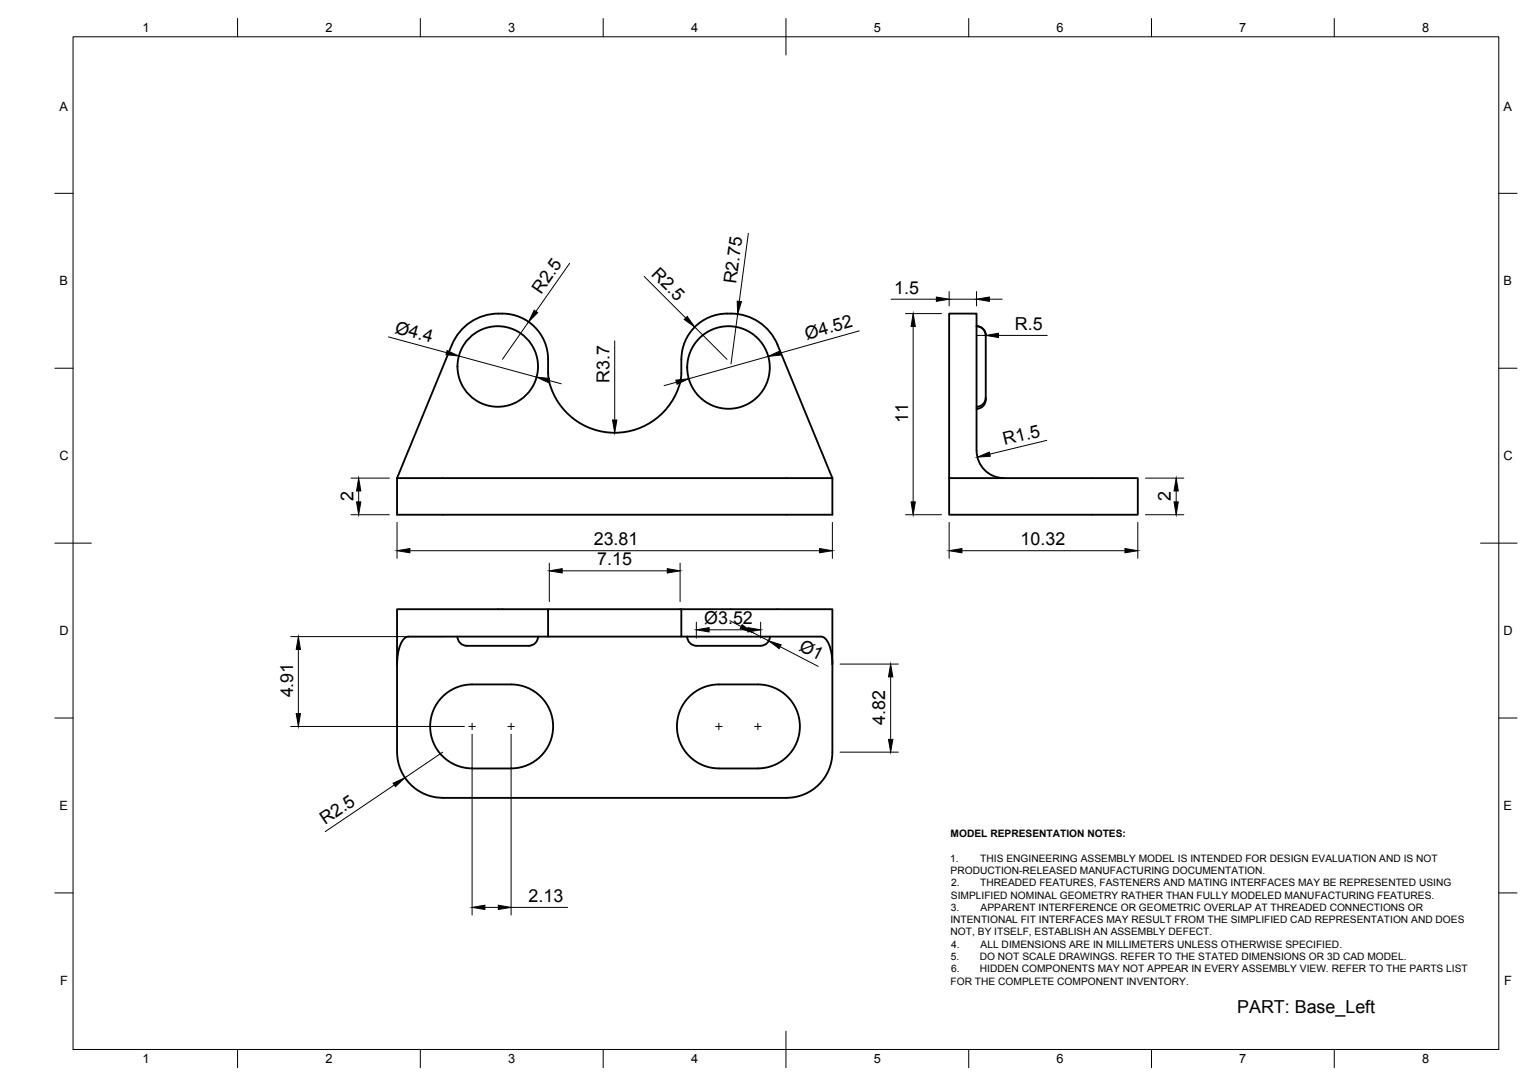
ISO-10303-21;
HEADER;
/* Generated by software containing ST-Developer
 * from STEP Tools, Inc. (www.steptools.com) 
 */

FILE_DESCRIPTION(
/* description */ (''),
/* implementation_level */ '2;1');

FILE_NAME(
/* name */ 'Base_Left.step',
/* time_stamp */ '2026-10-05T16:20:14-07:00',
/* author */ (''),
/* organization */ (''),
/* preprocessor_version */ 'ST-DEVELOPER v20.2',
/* originating_system */ 'Autodesk Translation Framework v15.15.0.0',
/* authorisation */ '');

FILE_SCHEMA (('AUTOMOTIVE_DESIGN { 1 0 10303 214 3 1 1 }'));
ENDSEC;

DATA;
#10=MECHANICAL_DESIGN_GEOMETRIC_PRESENTATION_REPRESENTATION('',(#248),#23577);
#207=ELLIPSE('',#4296,1.6218841056004,1.5);
#208=ELLIPSE('',#4297,1.6218841056004,1.5);
#213=TOROIDAL_SURFACE('',#4285,1.70133516896762,0.5);
#214=TOROIDAL_SURFACE('',#4290,1.75974879114541,0.5);
#230=SHAPE_REPRESENTATION_RELATIONSHIP('SRR','None',#23613,#239);
#239=ADVANCED_BREP_SHAPE_REPRESENTATION('',(#257),#23569);
#248=STYLED_ITEM('',(#23666),#257);
#257=MANIFOLD_SOLID_BREP('Body1',#4158);
#269=FACE_BOUND('',#640,.T.);
#270=FACE_BOUND('',#641,.T.);
#271=FACE_BOUND('',#670,.T.);
#272=FACE_BOUND('',#671,.T.);
#273=FACE_BOUND('',#673,.T.);
#274=FACE_BOUND('',#674,.T.);
#304=PLANE('',#4289);
#305=PLANE('',#4294);
#306=PLANE('',#4298);
#307=PLANE('',#4308);
#308=PLANE('',#4311);
#309=PLANE('',#4314);
#310=PLANE('',#4317);
#311=PLANE('',#4320);
#312=PLANE('',#4325);
#313=PLANE('',#4326);
#314=PLANE('',#4327);
#315=PLANE('',#4328);
#316=PLANE('',#4332);
#317=PLANE('',#4336);
#318=PLANE('',#4340);
#319=PLANE('',#4344);
#320=PLANE('',#4348);
#321=PLANE('',#4352);
#322=PLANE('',#4353);
#404=FACE_OUTER_BOUND('',#634,.T.);
#405=FACE_OUTER_BOUND('',#635,.T.);
#406=FACE_OUTER_BOUND('',#636,.T.);
#407=FACE_OUTER_BOUND('',#637,.T.);
#408=FACE_OUTER_BOUND('',#638,.T.);
#409=FACE_OUTER_BOUND('',#639,.T.);
#410=FACE_OUTER_BOUND('',#642,.T.);
#411=FACE_OUTER_BOUND('',#643,.T.);
#412=FACE_OUTER_BOUND('',#644,.T.);
#413=FACE_OUTER_BOUND('',#645,.T.);
#414=FACE_OUTER_BOUND('',#646,.T.);
#415=FACE_OUTER_BOUND('',#647,.T.);
#416=FACE_OUTER_BOUND('',#648,.T.);
#417=FACE_OUTER_BOUND('',#649,.T.);
#418=FACE_OUTER_BOUND('',#650,.T.);
#419=FACE_OUTER_BOUND('',#651,.T.);
#420=FACE_OUTER_BOUND('',#652,.T.);
#421=FACE_OUTER_BOUND('',#653,.T.);
#422=FACE_OUTER_BOUND('',#654,.T.);
#423=FACE_OUTER_BOUND('',#655,.T.);
#424=FACE_OUTER_BOUND('',#656,.T.);
#425=FACE_OUTER_BOUND('',#657,.T.);
#426=FACE_OUTER_BOUND('',#658,.T.);
#427=FACE_OUTER_BOUND('',#659,.T.);
#428=FACE_OUTER_BOUND('',#660,.T.);
#429=FACE_OUTER_BOUND('',#661,.T.);
#430=FACE_OUTER_BOUND('',#662,.T.);
#431=FACE_OUTER_BOUND('',#663,.T.);
#432=FACE_OUTER_BOUND('',#664,.T.);
#433=FACE_OUTER_BOUND('',#665,.T.);
#434=FACE_OUTER_BOUND('',#666,.T.);
#435=FACE_OUTER_BOUND('',#667,.T.);
#436=FACE_OUTER_BOUND('',#668,.T.);
#437=FACE_OUTER_BOUND('',#669,.T.);
#438=FACE_OUTER_BOUND('',#672,.T.);
#634=EDGE_LOOP('',(#2673,#2674,#2675,#2676));
#635=EDGE_LOOP('',(#2677));
#636=EDGE_LOOP('',(#2678,#2679,#2680,#2681));
#637=EDGE_LOOP('',(#2682));
#638=EDGE_LOOP('',(#2683,#2684,#2685,#2686));
#639=EDGE_LOOP('',(#2687,#2688,#2689,#2690,#2691,#2692,#2693,#2694,#2695,
#2696,#2697,#2698,#2699,#2700));
#640=EDGE_LOOP('',(#2701));
#641=EDGE_LOOP('',(#2702));
#642=EDGE_LOOP('',(#2703,#2704,#2705,#2706));
#643=EDGE_LOOP('',(#2707,#2708,#2709,#2710));
#644=EDGE_LOOP('',(#2711,#2712,#2713,#2714));
#645=EDGE_LOOP('',(#2715,#2716,#2717,#2718));
#646=EDGE_LOOP('',(#2719,#2720,#2721,#2722));
#647=EDGE_LOOP('',(#2723,#2724,#2725,#2726,#2727));
#648=EDGE_LOOP('',(#2728,#2729,#2730,#2731));
#649=EDGE_LOOP('',(#2732,#2733,#2734,#2735,#2736));
#650=EDGE_LOOP('',(#2737,#2738,#2739,#2740));
#651=EDGE_LOOP('',(#2741,#2742,#2743,#2744));
#652=EDGE_LOOP('',(#2745,#2746,#2747,#2748));
#653=EDGE_LOOP('',(#2749,#2750,#2751,#2752));
#654=EDGE_LOOP('',(#2753,#2754,#2755,#2756,#2757));
#655=EDGE_LOOP('',(#2758,#2759,#2760,#2761,#2762,#2763,#2764,#2765,#2766,
#2767,#2768,#2769,#2770,#2771,#2772,#2773));
#656=EDGE_LOOP('',(#2774,#2775,#2776,#2777));
#657=EDGE_LOOP('',(#2778,#2779,#2780,#2781));
#658=EDGE_LOOP('',(#2782,#2783,#2784,#2785));
#659=EDGE_LOOP('',(#2786,#2787,#2788,#2789));
#660=EDGE_LOOP('',(#2790,#2791,#2792,#2793));
#661=EDGE_LOOP('',(#2794,#2795,#2796,#2797));
#662=EDGE_LOOP('',(#2798,#2799,#2800,#2801));
#663=EDGE_LOOP('',(#2802,#2803,#2804,#2805));
#664=EDGE_LOOP('',(#2806,#2807,#2808,#2809));
#665=EDGE_LOOP('',(#2810,#2811,#2812,#2813,#2814));
#666=EDGE_LOOP('',(#2815,#2816,#2817,#2818));
#667=EDGE_LOOP('',(#2819,#2820,#2821,#2822));
#668=EDGE_LOOP('',(#2823,#2824,#2825,#2826));
#669=EDGE_LOOP('',(#2827,#2828,#2829,#2830,#2831,#2832));
#670=EDGE_LOOP('',(#2833,#2834,#2835,#2836));
#671=EDGE_LOOP('',(#2837,#2838,#2839,#2840));
#672=EDGE_LOOP('',(#2841,#2842,#2843,#2844,#2845,#2846));
#673=EDGE_LOOP('',(#2847,#2848,#2849,#2850));
#674=EDGE_LOOP('',(#2851,#2852,#2853,#2854));
#893=LINE('',#5835,#1178);
#894=LINE('',#5838,#1179);
#895=LINE('',#5841,#1180);
#896=LINE('',#5845,#1181);
#897=LINE('',#5849,#1182);
#898=LINE('',#5857,#1183);
#899=LINE('',#5861,#1184);
#900=LINE('',#5864,#1185);
#901=LINE('',#5867,#1186);
#902=LINE('',#5870,#1187);
#903=LINE('',#5873,#1188);
#904=LINE('',#5874,#1189);
#905=LINE('',#5879,#1190);
#906=LINE('',#5880,#1191);
#907=LINE('',#5883,#1192);
#908=LINE('',#5884,#1193);
#909=LINE('',#5888,#1194);
#910=LINE('',#5891,#1195);
#911=LINE('',#5892,#1196);
#912=LINE('',#5895,#1197);
#913=LINE('',#5898,#1198);
#914=LINE('',#5901,#1199);
#915=LINE('',#5902,#1200);
#916=LINE('',#5907,#1201);
#917=LINE('',#5908,#1202);
#918=LINE('',#5910,#1203);
#919=LINE('',#5914,#1204);
#920=LINE('',#5919,#1205);
#921=LINE('',#5921,#1206);
#922=LINE('',#5923,#1207);
#923=LINE('',#5924,#1208);
#924=LINE('',#5927,#1209);
#925=LINE('',#5928,#1210);
#926=LINE('',#5929,#1211);
#927=LINE('',#5934,#1212);
#928=LINE('',#5936,#1213);
#929=LINE('',#5938,#1214);
#930=LINE('',#5939,#1215);
#931=LINE('',#5945,#1216);
#932=LINE('',#5948,#1217);
#933=LINE('',#5950,#1218);
#934=LINE('',#5951,#1219);
#935=LINE('',#5958,#1220);
#936=LINE('',#5960,#1221);
#937=LINE('',#5962,#1222);
#938=LINE('',#5963,#1223);
#939=LINE('',#5969,#1224);
#940=LINE('',#5972,#1225);
#941=LINE('',#5974,#1226);
#942=LINE('',#5975,#1227);
#943=LINE('',#5981,#1228);
#944=LINE('',#5983,#1229);
#945=LINE('',#5984,#1230);
#946=LINE('',#5990,#1231);
#947=LINE('',#5993,#1232);
#948=LINE('',#5995,#1233);
#949=LINE('',#5996,#1234);
#1178=VECTOR('',#4746,10.);
#1179=VECTOR('',#4749,10.);
#1180=VECTOR('',#4752,9.99999999999999);
#1181=VECTOR('',#4755,10.);
#1182=VECTOR('',#4758,10.);
#1183=VECTOR('',#4765,10.);
#1184=VECTOR('',#4768,10.);
#1185=VECTOR('',#4771,9.99999999999999);
#1186=VECTOR('',#4774,10.);
#1187=VECTOR('',#4777,10.);
#1188=VECTOR('',#4780,10.);
#1189=VECTOR('',#4781,10.);
#1190=VECTOR('',#4786,10.);
#1191=VECTOR('',#4787,10.);
#1192=VECTOR('',#4790,10.);
#1193=VECTOR('',#4791,10.);
#1194=VECTOR('',#4796,10.);
#1195=VECTOR('',#4799,10.);
#1196=VECTOR('',#4800,9.99999999999999);
#1197=VECTOR('',#4803,10.);
#1198=VECTOR('',#4806,10.);
#1199=VECTOR('',#4809,9.99999999999999);
#1200=VECTOR('',#4810,10.);
#1201=VECTOR('',#4815,10.);
#1202=VECTOR('',#4816,10.);
#1203=VECTOR('',#4819,10.);
#1204=VECTOR('',#4824,10.);
#1205=VECTOR('',#4831,10.);
#1206=VECTOR('',#4832,10.);
#1207=VECTOR('',#4833,10.);
#1208=VECTOR('',#4834,10.);
#1209=VECTOR('',#4837,10.);
#1210=VECTOR('',#4838,10.);
#1211=VECTOR('',#4839,10.);
#1212=VECTOR('',#4844,10.);
#1213=VECTOR('',#4845,10.);
#1214=VECTOR('',#4846,10.);
#1215=VECTOR('',#4847,10.);
#1216=VECTOR('',#4854,10.);
#1217=VECTOR('',#4857,10.);
#1218=VECTOR('',#4858,10.);
#1219=VECTOR('',#4859,10.);
#1220=VECTOR('',#4868,10.);
#1221=VECTOR('',#4869,10.);
#1222=VECTOR('',#4870,10.);
#1223=VECTOR('',#4871,10.);
#1224=VECTOR('',#4878,10.);
#1225=VECTOR('',#4881,10.);
#1226=VECTOR('',#4882,10.);
#1227=VECTOR('',#4883,10.);
#1228=VECTOR('',#4892,10.);
#1229=VECTOR('',#4893,10.);
#1230=VECTOR('',#4894,10.);
#1231=VECTOR('',#4901,10.);
#1232=VECTOR('',#4904,10.);
#1233=VECTOR('',#4905,10.);
#1234=VECTOR('',#4906,10.);
#1461=CIRCLE('',#4286,1.70133516896762);
#1462=CIRCLE('',#4287,0.5);
#1463=CIRCLE('',#4288,2.20133516896762);
#1464=CIRCLE('',#4291,1.75974879114541);
#1465=CIRCLE('',#4292,0.5);
#1466=CIRCLE('',#4293,2.25974879114541);
#1467=CIRCLE('',#4299,2.75);
#1468=CIRCLE('',#4300,2.5);
#1469=CIRCLE('',#4301,2.00000000000029);
#1470=CIRCLE('',#4302,3.70283120062258);
#1471=CIRCLE('',#4303,2.00000000000029);
#1472=CIRCLE('',#4304,2.5);
#1473=CIRCLE('',#4305,2.75);
#1474=CIRCLE('',#4307,2.5);
#1475=CIRCLE('',#4310,2.5);
#1476=CIRCLE('',#4313,2.75);
#1477=CIRCLE('',#4316,2.75);
#1478=CIRCLE('',#4319,2.00000000000029);
#1479=CIRCLE('',#4322,2.00000000000029);
#1480=CIRCLE('',#4324,3.70283120062258);
#1481=CIRCLE('',#4330,2.29663666580012);
#1482=CIRCLE('',#4331,2.29663666580012);
#1483=CIRCLE('',#4334,2.29663666580012);
#1484=CIRCLE('',#4335,2.29663666580012);
#1485=CIRCLE('',#4338,2.29663666580012);
#1486=CIRCLE('',#4339,2.29663666580012);
#1487=CIRCLE('',#4342,2.29663666580012);
#1488=CIRCLE('',#4343,2.29663666580012);
#1489=CIRCLE('',#4346,2.50000000000001);
#1490=CIRCLE('',#4347,2.50000000000001);
#1491=CIRCLE('',#4350,2.5);
#1492=CIRCLE('',#4351,2.5);
#1640=VERTEX_POINT('',#5817);
#1641=VERTEX_POINT('',#5819);
#1642=VERTEX_POINT('',#5824);
#1643=VERTEX_POINT('',#5826);
#1644=VERTEX_POINT('',#5831);
#1645=VERTEX_POINT('',#5832);
#1646=VERTEX_POINT('',#5834);
#1647=VERTEX_POINT('',#5836);
#1648=VERTEX_POINT('',#5840);
#1649=VERTEX_POINT('',#5842);
#1650=VERTEX_POINT('',#5844);
#1651=VERTEX_POINT('',#5846);
#1652=VERTEX_POINT('',#5848);
#1653=VERTEX_POINT('',#5850);
#1654=VERTEX_POINT('',#5852);
#1655=VERTEX_POINT('',#5854);
#1656=VERTEX_POINT('',#5856);
#1657=VERTEX_POINT('',#5858);
#1658=VERTEX_POINT('',#5860);
#1659=VERTEX_POINT('',#5862);
#1660=VERTEX_POINT('',#5866);
#1661=VERTEX_POINT('',#5868);
#1662=VERTEX_POINT('',#5872);
#1663=VERTEX_POINT('',#5876);
#1664=VERTEX_POINT('',#5877);
#1665=VERTEX_POINT('',#5882);
#1666=VERTEX_POINT('',#5886);
#1667=VERTEX_POINT('',#5890);
#1668=VERTEX_POINT('',#5894);
#1669=VERTEX_POINT('',#5896);
#1670=VERTEX_POINT('',#5900);
#1671=VERTEX_POINT('',#5904);
#1672=VERTEX_POINT('',#5905);
#1673=VERTEX_POINT('',#5912);
#1674=VERTEX_POINT('',#5918);
#1675=VERTEX_POINT('',#5920);
#1676=VERTEX_POINT('',#5922);
#1677=VERTEX_POINT('',#5926);
#1678=VERTEX_POINT('',#5932);
#1679=VERTEX_POINT('',#5933);
#1680=VERTEX_POINT('',#5935);
#1681=VERTEX_POINT('',#5937);
#1682=VERTEX_POINT('',#5941);
#1683=VERTEX_POINT('',#5943);
#1684=VERTEX_POINT('',#5947);
#1685=VERTEX_POINT('',#5949);
#1686=VERTEX_POINT('',#5956);
#1687=VERTEX_POINT('',#5957);
#1688=VERTEX_POINT('',#5959);
#1689=VERTEX_POINT('',#5961);
#1690=VERTEX_POINT('',#5965);
#1691=VERTEX_POINT('',#5967);
#1692=VERTEX_POINT('',#5971);
#1693=VERTEX_POINT('',#5973);
#1694=VERTEX_POINT('',#5980);
#1695=VERTEX_POINT('',#5982);
#1696=VERTEX_POINT('',#5986);
#1697=VERTEX_POINT('',#5988);
#1698=VERTEX_POINT('',#5992);
#1699=VERTEX_POINT('',#5994);
#2053=EDGE_CURVE('',#1640,#1640,#1461,.T.);
#2054=EDGE_CURVE('',#1640,#1641,#1462,.T.);
#2055=EDGE_CURVE('',#1641,#1641,#1463,.T.);
#2056=EDGE_CURVE('',#1642,#1642,#1464,.T.);
#2057=EDGE_CURVE('',#1642,#1643,#1465,.T.);
#2058=EDGE_CURVE('',#1643,#1643,#1466,.T.);
#2059=EDGE_CURVE('',#1644,#1645,#207,.F.);
#2060=EDGE_CURVE('',#1644,#1646,#893,.T.);
#2061=EDGE_CURVE('',#1646,#1647,#208,.T.);
#2062=EDGE_CURVE('',#1647,#1645,#894,.T.);
#2063=EDGE_CURVE('',#1647,#1648,#895,.T.);
#2064=EDGE_CURVE('',#1649,#1648,#1467,.T.);
#2065=EDGE_CURVE('',#1650,#1649,#896,.T.);
#2066=EDGE_CURVE('',#1651,#1650,#1468,.T.);
#2067=EDGE_CURVE('',#1651,#1652,#897,.T.);
#2068=EDGE_CURVE('',#1652,#1653,#1469,.T.);
#2069=EDGE_CURVE('',#1653,#1654,#1470,.T.);
#2070=EDGE_CURVE('',#1654,#1655,#1471,.T.);
#2071=EDGE_CURVE('',#1655,#1656,#898,.T.);
#2072=EDGE_CURVE('',#1657,#1656,#1472,.T.);
#2073=EDGE_CURVE('',#1658,#1657,#899,.T.);
#2074=EDGE_CURVE('',#1659,#1658,#1473,.T.);
#2075=EDGE_CURVE('',#1659,#1645,#900,.T.);
#2076=EDGE_CURVE('',#1650,#1660,#901,.T.);
#2077=EDGE_CURVE('',#1660,#1661,#1474,.T.);
#2078=EDGE_CURVE('',#1661,#1651,#902,.T.);
#2079=EDGE_CURVE('',#1662,#1649,#903,.T.);
#2080=EDGE_CURVE('',#1662,#1660,#904,.T.);
#2081=EDGE_CURVE('',#1663,#1664,#1475,.T.);
#2082=EDGE_CURVE('',#1664,#1657,#905,.T.);
#2083=EDGE_CURVE('',#1656,#1663,#906,.T.);
#2084=EDGE_CURVE('',#1655,#1665,#907,.T.);
#2085=EDGE_CURVE('',#1663,#1665,#908,.T.);
#2086=EDGE_CURVE('',#1666,#1662,#1476,.T.);
#2087=EDGE_CURVE('',#1648,#1666,#909,.T.);
#2088=EDGE_CURVE('',#1646,#1667,#910,.T.);
#2089=EDGE_CURVE('',#1666,#1667,#911,.T.);
#2090=EDGE_CURVE('',#1658,#1668,#912,.T.);
#2091=EDGE_CURVE('',#1668,#1669,#1477,.T.);
#2092=EDGE_CURVE('',#1669,#1659,#913,.T.);
#2093=EDGE_CURVE('',#1670,#1669,#914,.T.);
#2094=EDGE_CURVE('',#1670,#1644,#915,.T.);
#2095=EDGE_CURVE('',#1671,#1672,#1478,.T.);
#2096=EDGE_CURVE('',#1653,#1671,#916,.T.);
#2097=EDGE_CURVE('',#1652,#1672,#917,.T.);
#2098=EDGE_CURVE('',#1672,#1661,#918,.T.);
#2099=EDGE_CURVE('',#1665,#1673,#1479,.T.);
#2100=EDGE_CURVE('',#1654,#1673,#919,.T.);
#2101=EDGE_CURVE('',#1673,#1671,#1480,.T.);
#2102=EDGE_CURVE('',#1674,#1646,#920,.T.);
#2103=EDGE_CURVE('',#1675,#1674,#921,.T.);
#2104=EDGE_CURVE('',#1676,#1675,#922,.T.);
#2105=EDGE_CURVE('',#1676,#1667,#923,.T.);
#2106=EDGE_CURVE('',#1676,#1677,#924,.T.);
#2107=EDGE_CURVE('',#1677,#1670,#925,.T.);
#2108=EDGE_CURVE('',#1664,#1668,#926,.T.);
#2109=EDGE_CURVE('',#1678,#1679,#927,.T.);
#2110=EDGE_CURVE('',#1679,#1680,#928,.T.);
#2111=EDGE_CURVE('',#1681,#1680,#929,.T.);
#2112=EDGE_CURVE('',#1678,#1681,#930,.T.);
#2113=EDGE_CURVE('',#1682,#1678,#1481,.T.);
#2114=EDGE_CURVE('',#1683,#1681,#1482,.T.);
#2115=EDGE_CURVE('',#1682,#1683,#931,.T.);
#2116=EDGE_CURVE('',#1684,#1682,#932,.T.);
#2117=EDGE_CURVE('',#1685,#1683,#933,.T.);
#2118=EDGE_CURVE('',#1684,#1685,#934,.T.);
#2119=EDGE_CURVE('',#1679,#1684,#1483,.T.);
#2120=EDGE_CURVE('',#1680,#1685,#1484,.T.);
#2121=EDGE_CURVE('',#1686,#1687,#935,.T.);
#2122=EDGE_CURVE('',#1687,#1688,#936,.T.);
#2123=EDGE_CURVE('',#1689,#1688,#937,.T.);
#2124=EDGE_CURVE('',#1686,#1689,#938,.T.);
#2125=EDGE_CURVE('',#1690,#1686,#1485,.T.);
#2126=EDGE_CURVE('',#1691,#1689,#1486,.T.);
#2127=EDGE_CURVE('',#1690,#1691,#939,.T.);
#2128=EDGE_CURVE('',#1692,#1690,#940,.T.);
#2129=EDGE_CURVE('',#1693,#1691,#941,.T.);
#2130=EDGE_CURVE('',#1692,#1693,#942,.T.);
#2131=EDGE_CURVE('',#1687,#1692,#1487,.T.);
#2132=EDGE_CURVE('',#1688,#1693,#1488,.T.);
#2133=EDGE_CURVE('',#1677,#1694,#943,.T.);
#2134=EDGE_CURVE('',#1694,#1695,#944,.T.);
#2135=EDGE_CURVE('',#1644,#1695,#945,.T.);
#2136=EDGE_CURVE('',#1696,#1675,#1489,.T.);
#2137=EDGE_CURVE('',#1697,#1674,#1490,.T.);
#2138=EDGE_CURVE('',#1696,#1697,#946,.T.);
#2139=EDGE_CURVE('',#1696,#1698,#947,.T.);
#2140=EDGE_CURVE('',#1699,#1697,#948,.T.);
#2141=EDGE_CURVE('',#1698,#1699,#949,.T.);
#2142=EDGE_CURVE('',#1694,#1698,#1491,.T.);
#2143=EDGE_CURVE('',#1695,#1699,#1492,.T.);
#2673=ORIENTED_EDGE('',*,*,#2053,.T.);
#2674=ORIENTED_EDGE('',*,*,#2054,.T.);
#2675=ORIENTED_EDGE('',*,*,#2055,.F.);
#2676=ORIENTED_EDGE('',*,*,#2054,.F.);
#2677=ORIENTED_EDGE('',*,*,#2053,.F.);
#2678=ORIENTED_EDGE('',*,*,#2056,.T.);
#2679=ORIENTED_EDGE('',*,*,#2057,.T.);
#2680=ORIENTED_EDGE('',*,*,#2058,.F.);
#2681=ORIENTED_EDGE('',*,*,#2057,.F.);
#2682=ORIENTED_EDGE('',*,*,#2056,.F.);
#2683=ORIENTED_EDGE('',*,*,#2059,.F.);
#2684=ORIENTED_EDGE('',*,*,#2060,.T.);
#2685=ORIENTED_EDGE('',*,*,#2061,.T.);
#2686=ORIENTED_EDGE('',*,*,#2062,.T.);
#2687=ORIENTED_EDGE('',*,*,#2062,.F.);
#2688=ORIENTED_EDGE('',*,*,#2063,.T.);
#2689=ORIENTED_EDGE('',*,*,#2064,.F.);
#2690=ORIENTED_EDGE('',*,*,#2065,.F.);
#2691=ORIENTED_EDGE('',*,*,#2066,.F.);
#2692=ORIENTED_EDGE('',*,*,#2067,.T.);
#2693=ORIENTED_EDGE('',*,*,#2068,.T.);
#2694=ORIENTED_EDGE('',*,*,#2069,.T.);
#2695=ORIENTED_EDGE('',*,*,#2070,.T.);
#2696=ORIENTED_EDGE('',*,*,#2071,.T.);
#2697=ORIENTED_EDGE('',*,*,#2072,.F.);
#2698=ORIENTED_EDGE('',*,*,#2073,.F.);
#2699=ORIENTED_EDGE('',*,*,#2074,.F.);
#2700=ORIENTED_EDGE('',*,*,#2075,.T.);
#2701=ORIENTED_EDGE('',*,*,#2055,.T.);
#2702=ORIENTED_EDGE('',*,*,#2058,.T.);
#2703=ORIENTED_EDGE('',*,*,#2066,.T.);
#2704=ORIENTED_EDGE('',*,*,#2076,.T.);
#2705=ORIENTED_EDGE('',*,*,#2077,.T.);
#2706=ORIENTED_EDGE('',*,*,#2078,.T.);
#2707=ORIENTED_EDGE('',*,*,#2076,.F.);
#2708=ORIENTED_EDGE('',*,*,#2065,.T.);
#2709=ORIENTED_EDGE('',*,*,#2079,.F.);
#2710=ORIENTED_EDGE('',*,*,#2080,.T.);
#2711=ORIENTED_EDGE('',*,*,#2081,.T.);
#2712=ORIENTED_EDGE('',*,*,#2082,.T.);
#2713=ORIENTED_EDGE('',*,*,#2072,.T.);
#2714=ORIENTED_EDGE('',*,*,#2083,.T.);
#2715=ORIENTED_EDGE('',*,*,#2083,.F.);
#2716=ORIENTED_EDGE('',*,*,#2071,.F.);
#2717=ORIENTED_EDGE('',*,*,#2084,.T.);
#2718=ORIENTED_EDGE('',*,*,#2085,.F.);
#2719=ORIENTED_EDGE('',*,*,#2086,.T.);
#2720=ORIENTED_EDGE('',*,*,#2079,.T.);
#2721=ORIENTED_EDGE('',*,*,#2064,.T.);
#2722=ORIENTED_EDGE('',*,*,#2087,.T.);
#2723=ORIENTED_EDGE('',*,*,#2087,.F.);
#2724=ORIENTED_EDGE('',*,*,#2063,.F.);
#2725=ORIENTED_EDGE('',*,*,#2061,.F.);
#2726=ORIENTED_EDGE('',*,*,#2088,.T.);
#2727=ORIENTED_EDGE('',*,*,#2089,.F.);
#2728=ORIENTED_EDGE('',*,*,#2074,.T.);
#2729=ORIENTED_EDGE('',*,*,#2090,.T.);
#2730=ORIENTED_EDGE('',*,*,#2091,.T.);
#2731=ORIENTED_EDGE('',*,*,#2092,.T.);
#2732=ORIENTED_EDGE('',*,*,#2092,.F.);
#2733=ORIENTED_EDGE('',*,*,#2093,.F.);
#2734=ORIENTED_EDGE('',*,*,#2094,.T.);
#2735=ORIENTED_EDGE('',*,*,#2059,.T.);
#2736=ORIENTED_EDGE('',*,*,#2075,.F.);
#2737=ORIENTED_EDGE('',*,*,#2095,.F.);
#2738=ORIENTED_EDGE('',*,*,#2096,.F.);
#2739=ORIENTED_EDGE('',*,*,#2068,.F.);
#2740=ORIENTED_EDGE('',*,*,#2097,.T.);
#2741=ORIENTED_EDGE('',*,*,#2078,.F.);
#2742=ORIENTED_EDGE('',*,*,#2098,.F.);
#2743=ORIENTED_EDGE('',*,*,#2097,.F.);
#2744=ORIENTED_EDGE('',*,*,#2067,.F.);
#2745=ORIENTED_EDGE('',*,*,#2099,.F.);
#2746=ORIENTED_EDGE('',*,*,#2084,.F.);
#2747=ORIENTED_EDGE('',*,*,#2070,.F.);
#2748=ORIENTED_EDGE('',*,*,#2100,.T.);
#2749=ORIENTED_EDGE('',*,*,#2101,.F.);
#2750=ORIENTED_EDGE('',*,*,#2100,.F.);
#2751=ORIENTED_EDGE('',*,*,#2069,.F.);
#2752=ORIENTED_EDGE('',*,*,#2096,.T.);
#2753=ORIENTED_EDGE('',*,*,#2088,.F.);
#2754=ORIENTED_EDGE('',*,*,#2102,.F.);
#2755=ORIENTED_EDGE('',*,*,#2103,.F.);
#2756=ORIENTED_EDGE('',*,*,#2104,.F.);
#2757=ORIENTED_EDGE('',*,*,#2105,.T.);
#2758=ORIENTED_EDGE('',*,*,#2077,.F.);
#2759=ORIENTED_EDGE('',*,*,#2080,.F.);
#2760=ORIENTED_EDGE('',*,*,#2086,.F.);
#2761=ORIENTED_EDGE('',*,*,#2089,.T.);
#2762=ORIENTED_EDGE('',*,*,#2105,.F.);
#2763=ORIENTED_EDGE('',*,*,#2106,.T.);
#2764=ORIENTED_EDGE('',*,*,#2107,.T.);
#2765=ORIENTED_EDGE('',*,*,#2093,.T.);
#2766=ORIENTED_EDGE('',*,*,#2091,.F.);
#2767=ORIENTED_EDGE('',*,*,#2108,.F.);
#2768=ORIENTED_EDGE('',*,*,#2081,.F.);
#2769=ORIENTED_EDGE('',*,*,#2085,.T.);
#2770=ORIENTED_EDGE('',*,*,#2099,.T.);
#2771=ORIENTED_EDGE('',*,*,#2101,.T.);
#2772=ORIENTED_EDGE('',*,*,#2095,.T.);
#2773=ORIENTED_EDGE('',*,*,#2098,.T.);
#2774=ORIENTED_EDGE('',*,*,#2082,.F.);
#2775=ORIENTED_EDGE('',*,*,#2108,.T.);
#2776=ORIENTED_EDGE('',*,*,#2090,.F.);
#2777=ORIENTED_EDGE('',*,*,#2073,.T.);
#2778=ORIENTED_EDGE('',*,*,#2109,.T.);
#2779=ORIENTED_EDGE('',*,*,#2110,.T.);
#2780=ORIENTED_EDGE('',*,*,#2111,.F.);
#2781=ORIENTED_EDGE('',*,*,#2112,.F.);
#2782=ORIENTED_EDGE('',*,*,#2113,.T.);
#2783=ORIENTED_EDGE('',*,*,#2112,.T.);
#2784=ORIENTED_EDGE('',*,*,#2114,.F.);
#2785=ORIENTED_EDGE('',*,*,#2115,.F.);
#2786=ORIENTED_EDGE('',*,*,#2116,.T.);
#2787=ORIENTED_EDGE('',*,*,#2115,.T.);
#2788=ORIENTED_EDGE('',*,*,#2117,.F.);
#2789=ORIENTED_EDGE('',*,*,#2118,.F.);
#2790=ORIENTED_EDGE('',*,*,#2119,.T.);
#2791=ORIENTED_EDGE('',*,*,#2118,.T.);
#2792=ORIENTED_EDGE('',*,*,#2120,.F.);
#2793=ORIENTED_EDGE('',*,*,#2110,.F.);
#2794=ORIENTED_EDGE('',*,*,#2121,.T.);
#2795=ORIENTED_EDGE('',*,*,#2122,.T.);
#2796=ORIENTED_EDGE('',*,*,#2123,.F.);
#2797=ORIENTED_EDGE('',*,*,#2124,.F.);
#2798=ORIENTED_EDGE('',*,*,#2125,.T.);
#2799=ORIENTED_EDGE('',*,*,#2124,.T.);
#2800=ORIENTED_EDGE('',*,*,#2126,.F.);
#2801=ORIENTED_EDGE('',*,*,#2127,.F.);
#2802=ORIENTED_EDGE('',*,*,#2128,.T.);
#2803=ORIENTED_EDGE('',*,*,#2127,.T.);
#2804=ORIENTED_EDGE('',*,*,#2129,.F.);
#2805=ORIENTED_EDGE('',*,*,#2130,.F.);
#2806=ORIENTED_EDGE('',*,*,#2131,.T.);
#2807=ORIENTED_EDGE('',*,*,#2130,.T.);
#2808=ORIENTED_EDGE('',*,*,#2132,.F.);
#2809=ORIENTED_EDGE('',*,*,#2122,.F.);
#2810=ORIENTED_EDGE('',*,*,#2094,.F.);
#2811=ORIENTED_EDGE('',*,*,#2107,.F.);
#2812=ORIENTED_EDGE('',*,*,#2133,.T.);
#2813=ORIENTED_EDGE('',*,*,#2134,.T.);
#2814=ORIENTED_EDGE('',*,*,#2135,.F.);
#2815=ORIENTED_EDGE('',*,*,#2136,.T.);
#2816=ORIENTED_EDGE('',*,*,#2103,.T.);
#2817=ORIENTED_EDGE('',*,*,#2137,.F.);
#2818=ORIENTED_EDGE('',*,*,#2138,.F.);
#2819=ORIENTED_EDGE('',*,*,#2139,.F.);
#2820=ORIENTED_EDGE('',*,*,#2138,.T.);
#2821=ORIENTED_EDGE('',*,*,#2140,.F.);
#2822=ORIENTED_EDGE('',*,*,#2141,.F.);
#2823=ORIENTED_EDGE('',*,*,#2142,.T.);
#2824=ORIENTED_EDGE('',*,*,#2141,.T.);
#2825=ORIENTED_EDGE('',*,*,#2143,.F.);
#2826=ORIENTED_EDGE('',*,*,#2134,.F.);
#2827=ORIENTED_EDGE('',*,*,#2060,.F.);
#2828=ORIENTED_EDGE('',*,*,#2135,.T.);
#2829=ORIENTED_EDGE('',*,*,#2143,.T.);
#2830=ORIENTED_EDGE('',*,*,#2140,.T.);
#2831=ORIENTED_EDGE('',*,*,#2137,.T.);
#2832=ORIENTED_EDGE('',*,*,#2102,.T.);
#2833=ORIENTED_EDGE('',*,*,#2132,.T.);
#2834=ORIENTED_EDGE('',*,*,#2129,.T.);
#2835=ORIENTED_EDGE('',*,*,#2126,.T.);
#2836=ORIENTED_EDGE('',*,*,#2123,.T.);
#2837=ORIENTED_EDGE('',*,*,#2120,.T.);
#2838=ORIENTED_EDGE('',*,*,#2117,.T.);
#2839=ORIENTED_EDGE('',*,*,#2114,.T.);
#2840=ORIENTED_EDGE('',*,*,#2111,.T.);
#2841=ORIENTED_EDGE('',*,*,#2142,.F.);
#2842=ORIENTED_EDGE('',*,*,#2133,.F.);
#2843=ORIENTED_EDGE('',*,*,#2106,.F.);
#2844=ORIENTED_EDGE('',*,*,#2104,.T.);
#2845=ORIENTED_EDGE('',*,*,#2136,.F.);
#2846=ORIENTED_EDGE('',*,*,#2139,.T.);
#2847=ORIENTED_EDGE('',*,*,#2131,.F.);
#2848=ORIENTED_EDGE('',*,*,#2121,.F.);
#2849=ORIENTED_EDGE('',*,*,#2125,.F.);
#2850=ORIENTED_EDGE('',*,*,#2128,.F.);
#2851=ORIENTED_EDGE('',*,*,#2119,.F.);
#2852=ORIENTED_EDGE('',*,*,#2109,.F.);
#2853=ORIENTED_EDGE('',*,*,#2113,.F.);
#2854=ORIENTED_EDGE('',*,*,#2116,.F.);
#3845=CYLINDRICAL_SURFACE('',#4295,1.5);
#3846=CYLINDRICAL_SURFACE('',#4306,2.5);
#3847=CYLINDRICAL_SURFACE('',#4309,2.5);
#3848=CYLINDRICAL_SURFACE('',#4312,2.75);
#3849=CYLINDRICAL_SURFACE('',#4315,2.75);
#3850=CYLINDRICAL_SURFACE('',#4318,2.00000000000029);
#3851=CYLINDRICAL_SURFACE('',#4321,2.00000000000029);
#3852=CYLINDRICAL_SURFACE('',#4323,3.70283120062258);
#3853=CYLINDRICAL_SURFACE('',#4329,2.29663666580012);
#3854=CYLINDRICAL_SURFACE('',#4333,2.29663666580012);
#3855=CYLINDRICAL_SURFACE('',#4337,2.29663666580012);
#3856=CYLINDRICAL_SURFACE('',#4341,2.29663666580012);
#3857=CYLINDRICAL_SURFACE('',#4345,2.50000000000001);
#3858=CYLINDRICAL_SURFACE('',#4349,2.5);
#3939=ADVANCED_FACE('',(#404),#213,.T.);
#3940=ADVANCED_FACE('',(#405),#304,.T.);
#3941=ADVANCED_FACE('',(#406),#214,.T.);
#3942=ADVANCED_FACE('',(#407),#305,.T.);
#3943=ADVANCED_FACE('',(#408),#3845,.F.);
#3944=ADVANCED_FACE('',(#409,#269,#270),#306,.T.);
#3945=ADVANCED_FACE('',(#410),#3846,.T.);
#3946=ADVANCED_FACE('',(#411),#307,.T.);
#3947=ADVANCED_FACE('',(#412),#3847,.T.);
#3948=ADVANCED_FACE('',(#413),#308,.F.);
#3949=ADVANCED_FACE('',(#414),#3848,.T.);
#3950=ADVANCED_FACE('',(#415),#309,.F.);
#3951=ADVANCED_FACE('',(#416),#3849,.T.);
#3952=ADVANCED_FACE('',(#417),#310,.F.);
#3953=ADVANCED_FACE('',(#418),#3850,.F.);
#3954=ADVANCED_FACE('',(#419),#311,.F.);
#3955=ADVANCED_FACE('',(#420),#3851,.F.);
#3956=ADVANCED_FACE('',(#421),#3852,.F.);
#3957=ADVANCED_FACE('',(#422),#312,.T.);
#3958=ADVANCED_FACE('',(#423),#313,.T.);
#3959=ADVANCED_FACE('',(#424),#314,.T.);
#3960=ADVANCED_FACE('',(#425),#315,.T.);
#3961=ADVANCED_FACE('',(#426),#3853,.F.);
#3962=ADVANCED_FACE('',(#427),#316,.T.);
#3963=ADVANCED_FACE('',(#428),#3854,.F.);
#3964=ADVANCED_FACE('',(#429),#317,.T.);
#3965=ADVANCED_FACE('',(#430),#3855,.F.);
#3966=ADVANCED_FACE('',(#431),#318,.T.);
#3967=ADVANCED_FACE('',(#432),#3856,.F.);
#3968=ADVANCED_FACE('',(#433),#319,.T.);
#3969=ADVANCED_FACE('',(#434),#3857,.T.);
#3970=ADVANCED_FACE('',(#435),#320,.T.);
#3971=ADVANCED_FACE('',(#436),#3858,.T.);
#3972=ADVANCED_FACE('',(#437,#271,#272),#321,.T.);
#3973=ADVANCED_FACE('',(#438,#273,#274),#322,.F.);
#4158=CLOSED_SHELL('',(#3939,#3940,#3941,#3942,#3943,#3944,#3945,#3946,
#3947,#3948,#3949,#3950,#3951,#3952,#3953,#3954,#3955,#3956,#3957,#3958,
#3959,#3960,#3961,#3962,#3963,#3964,#3965,#3966,#3967,#3968,#3969,#3970,
#3971,#3972,#3973));
#4284=AXIS2_PLACEMENT_3D('',#5815,#4720,#4721);
#4285=AXIS2_PLACEMENT_3D('',#5816,#4722,#4723);
#4286=AXIS2_PLACEMENT_3D('',#5818,#4724,#4725);
#4287=AXIS2_PLACEMENT_3D('',#5820,#4726,#4727);
#4288=AXIS2_PLACEMENT_3D('',#5821,#4728,#4729);
#4289=AXIS2_PLACEMENT_3D('',#5822,#4730,#4731);
#4290=AXIS2_PLACEMENT_3D('',#5823,#4732,#4733);
#4291=AXIS2_PLACEMENT_3D('',#5825,#4734,#4735);
#4292=AXIS2_PLACEMENT_3D('',#5827,#4736,#4737);
#4293=AXIS2_PLACEMENT_3D('',#5828,#4738,#4739);
#4294=AXIS2_PLACEMENT_3D('',#5829,#4740,#4741);
#4295=AXIS2_PLACEMENT_3D('',#5830,#4742,#4743);
#4296=AXIS2_PLACEMENT_3D('',#5833,#4744,#4745);
#4297=AXIS2_PLACEMENT_3D('',#5837,#4747,#4748);
#4298=AXIS2_PLACEMENT_3D('',#5839,#4750,#4751);
#4299=AXIS2_PLACEMENT_3D('',#5843,#4753,#4754);
#4300=AXIS2_PLACEMENT_3D('',#5847,#4756,#4757);
#4301=AXIS2_PLACEMENT_3D('',#5851,#4759,#4760);
#4302=AXIS2_PLACEMENT_3D('',#5853,#4761,#4762);
#4303=AXIS2_PLACEMENT_3D('',#5855,#4763,#4764);
#4304=AXIS2_PLACEMENT_3D('',#5859,#4766,#4767);
#4305=AXIS2_PLACEMENT_3D('',#5863,#4769,#4770);
#4306=AXIS2_PLACEMENT_3D('',#5865,#4772,#4773);
#4307=AXIS2_PLACEMENT_3D('',#5869,#4775,#4776);
#4308=AXIS2_PLACEMENT_3D('',#5871,#4778,#4779);
#4309=AXIS2_PLACEMENT_3D('',#5875,#4782,#4783);
#4310=AXIS2_PLACEMENT_3D('',#5878,#4784,#4785);
#4311=AXIS2_PLACEMENT_3D('',#5881,#4788,#4789);
#4312=AXIS2_PLACEMENT_3D('',#5885,#4792,#4793);
#4313=AXIS2_PLACEMENT_3D('',#5887,#4794,#4795);
#4314=AXIS2_PLACEMENT_3D('',#5889,#4797,#4798);
#4315=AXIS2_PLACEMENT_3D('',#5893,#4801,#4802);
#4316=AXIS2_PLACEMENT_3D('',#5897,#4804,#4805);
#4317=AXIS2_PLACEMENT_3D('',#5899,#4807,#4808);
#4318=AXIS2_PLACEMENT_3D('',#5903,#4811,#4812);
#4319=AXIS2_PLACEMENT_3D('',#5906,#4813,#4814);
#4320=AXIS2_PLACEMENT_3D('',#5909,#4817,#4818);
#4321=AXIS2_PLACEMENT_3D('',#5911,#4820,#4821);
#4322=AXIS2_PLACEMENT_3D('',#5913,#4822,#4823);
#4323=AXIS2_PLACEMENT_3D('',#5915,#4825,#4826);
#4324=AXIS2_PLACEMENT_3D('',#5916,#4827,#4828);
#4325=AXIS2_PLACEMENT_3D('',#5917,#4829,#4830);
#4326=AXIS2_PLACEMENT_3D('',#5925,#4835,#4836);
#4327=AXIS2_PLACEMENT_3D('',#5930,#4840,#4841);
#4328=AXIS2_PLACEMENT_3D('',#5931,#4842,#4843);
#4329=AXIS2_PLACEMENT_3D('',#5940,#4848,#4849);
#4330=AXIS2_PLACEMENT_3D('',#5942,#4850,#4851);
#4331=AXIS2_PLACEMENT_3D('',#5944,#4852,#4853);
#4332=AXIS2_PLACEMENT_3D('',#5946,#4855,#4856);
#4333=AXIS2_PLACEMENT_3D('',#5952,#4860,#4861);
#4334=AXIS2_PLACEMENT_3D('',#5953,#4862,#4863);
#4335=AXIS2_PLACEMENT_3D('',#5954,#4864,#4865);
#4336=AXIS2_PLACEMENT_3D('',#5955,#4866,#4867);
#4337=AXIS2_PLACEMENT_3D('',#5964,#4872,#4873);
#4338=AXIS2_PLACEMENT_3D('',#5966,#4874,#4875);
#4339=AXIS2_PLACEMENT_3D('',#5968,#4876,#4877);
#4340=AXIS2_PLACEMENT_3D('',#5970,#4879,#4880);
#4341=AXIS2_PLACEMENT_3D('',#5976,#4884,#4885);
#4342=AXIS2_PLACEMENT_3D('',#5977,#4886,#4887);
#4343=AXIS2_PLACEMENT_3D('',#5978,#4888,#4889);
#4344=AXIS2_PLACEMENT_3D('',#5979,#4890,#4891);
#4345=AXIS2_PLACEMENT_3D('',#5985,#4895,#4896);
#4346=AXIS2_PLACEMENT_3D('',#5987,#4897,#4898);
#4347=AXIS2_PLACEMENT_3D('',#5989,#4899,#4900);
#4348=AXIS2_PLACEMENT_3D('',#5991,#4902,#4903);
#4349=AXIS2_PLACEMENT_3D('',#5997,#4907,#4908);
#4350=AXIS2_PLACEMENT_3D('',#5998,#4909,#4910);
#4351=AXIS2_PLACEMENT_3D('',#5999,#4911,#4912);
#4352=AXIS2_PLACEMENT_3D('',#6000,#4913,#4914);
#4353=AXIS2_PLACEMENT_3D('',#6001,#4915,#4916);
#4720=DIRECTION('axis',(0.,0.,1.));
#4721=DIRECTION('refdir',(1.,0.,0.));
#4722=DIRECTION('center_axis',(0.,-1.,0.));
#4723=DIRECTION('ref_axis',(0.,0.,-1.));
#4724=DIRECTION('center_axis',(0.,1.,0.));
#4725=DIRECTION('ref_axis',(1.,0.,0.));
#4726=DIRECTION('center_axis',(-1.,0.,0.));
#4727=DIRECTION('ref_axis',(0.,0.,1.));
#4728=DIRECTION('center_axis',(0.,1.,0.));
#4729=DIRECTION('ref_axis',(0.,0.,-1.));
#4730=DIRECTION('center_axis',(0.,-1.,0.));
#4731=DIRECTION('ref_axis',(1.,0.,0.));
#4732=DIRECTION('center_axis',(0.,-1.,0.));
#4733=DIRECTION('ref_axis',(0.,0.,-1.));
#4734=DIRECTION('center_axis',(0.,1.,0.));
#4735=DIRECTION('ref_axis',(1.,0.,0.));
#4736=DIRECTION('center_axis',(-1.,0.,0.));
#4737=DIRECTION('ref_axis',(0.,0.,1.));
#4738=DIRECTION('center_axis',(0.,1.,0.));
#4739=DIRECTION('ref_axis',(0.,0.,-1.));
#4740=DIRECTION('center_axis',(0.,-1.,0.));
#4741=DIRECTION('ref_axis',(1.,0.,0.));
#4742=DIRECTION('center_axis',(-1.,0.,0.));
#4743=DIRECTION('ref_axis',(0.,0.707106781186547,-0.707106781186548));
#4744=DIRECTION('center_axis',(-0.924850298995146,0.,0.380331335086382));
#4745=DIRECTION('ref_axis',(-0.380331335086382,-3.4226336542529E-16,-0.924850298995146));
#4746=DIRECTION('',(1.,0.,0.));
#4747=DIRECTION('center_axis',(0.924850298995146,0.,0.380331335086382));
#4748=DIRECTION('ref_axis',(0.380331335086382,0.,-0.924850298995146));
#4749=DIRECTION('',(-1.,0.,0.));
#4750=DIRECTION('center_axis',(0.,-1.,0.));
#4751=DIRECTION('ref_axis',(1.,0.,0.));
#4752=DIRECTION('',(-0.380331335086382,0.,0.924850298995146));
#4753=DIRECTION('center_axis',(0.,1.,0.));
#4754=DIRECTION('ref_axis',(0.556627642555425,0.,0.830762100449455));
#4755=DIRECTION('',(1.,0.,0.));
#4756=DIRECTION('center_axis',(0.,1.,0.));
#4757=DIRECTION('ref_axis',(-0.707106781186548,0.,0.707106781186548));
#4758=DIRECTION('',(0.,0.,-1.));
#4759=DIRECTION('center_axis',(0.,1.,0.));
#4760=DIRECTION('ref_axis',(0.965748659616483,0.,-0.259479337229319));
#4761=DIRECTION('center_axis',(0.,1.,0.));
#4762=DIRECTION('ref_axis',(-0.965748659616478,0.,-0.259479337229339));
#4763=DIRECTION('center_axis',(0.,1.,0.));
#4764=DIRECTION('ref_axis',(-1.,0.,-1.85962356624686E-14));
#4765=DIRECTION('',(0.,0.,1.));
#4766=DIRECTION('center_axis',(0.,1.,0.));
#4767=DIRECTION('ref_axis',(0.707106781186548,0.,0.707106781186548));
#4768=DIRECTION('',(1.,0.,0.));
#4769=DIRECTION('center_axis',(0.,1.,0.));
#4770=DIRECTION('ref_axis',(-0.556627642555424,0.,0.830762100449455));
#4771=DIRECTION('',(-0.380331335086382,0.,-0.924850298995146));
#4772=DIRECTION('center_axis',(0.,-1.,0.));
#4773=DIRECTION('ref_axis',(-0.707106781186548,0.,0.707106781186548));
#4774=DIRECTION('',(0.,1.,0.));
#4775=DIRECTION('center_axis',(0.,-1.,0.));
#4776=DIRECTION('ref_axis',(-0.707106781186548,0.,0.707106781186548));
#4777=DIRECTION('',(0.,-1.,0.));
#4778=DIRECTION('center_axis',(0.,0.,1.));
#4779=DIRECTION('ref_axis',(1.,0.,0.));
#4780=DIRECTION('',(0.,-1.,0.));
#4781=DIRECTION('',(-1.,0.,0.));
#4782=DIRECTION('center_axis',(0.,1.,0.));
#4783=DIRECTION('ref_axis',(0.707106781186548,0.,0.707106781186548));
#4784=DIRECTION('center_axis',(0.,-1.,0.));
#4785=DIRECTION('ref_axis',(0.707106781186548,0.,0.707106781186548));
#4786=DIRECTION('',(0.,-1.,0.));
#4787=DIRECTION('',(0.,1.,0.));
#4788=DIRECTION('center_axis',(-1.,0.,0.));
#4789=DIRECTION('ref_axis',(0.,0.,1.));
#4790=DIRECTION('',(0.,1.,0.));
#4791=DIRECTION('',(0.,0.,-1.));
#4792=DIRECTION('center_axis',(0.,1.,0.));
#4793=DIRECTION('ref_axis',(0.556627642555425,0.,0.830762100449455));
#4794=DIRECTION('center_axis',(0.,-1.,0.));
#4795=DIRECTION('ref_axis',(0.556627642555425,0.,0.830762100449455));
#4796=DIRECTION('',(0.,1.,0.));
#4797=DIRECTION('center_axis',(-0.924850298995146,0.,-0.380331335086382));
#4798=DIRECTION('ref_axis',(-0.380331335086382,0.,0.924850298995145));
#4799=DIRECTION('',(0.,1.,0.));
#4800=DIRECTION('',(0.380331335086382,0.,-0.924850298995146));
#4801=DIRECTION('center_axis',(0.,-1.,0.));
#4802=DIRECTION('ref_axis',(-0.556627642555424,0.,0.830762100449455));
#4803=DIRECTION('',(0.,1.,0.));
#4804=DIRECTION('center_axis',(0.,-1.,0.));
#4805=DIRECTION('ref_axis',(-0.556627642555424,0.,0.830762100449455));
#4806=DIRECTION('',(0.,-1.,0.));
#4807=DIRECTION('center_axis',(0.924850298995146,0.,-0.380331335086382));
#4808=DIRECTION('ref_axis',(-0.380331335086382,0.,-0.924850298995145));
#4809=DIRECTION('',(0.380331335086382,0.,0.924850298995146));
#4810=DIRECTION('',(3.51417407375166E-16,-1.,0.));
#4811=DIRECTION('center_axis',(0.,1.,0.));
#4812=DIRECTION('ref_axis',(0.965748659616483,0.,-0.259479337229319));
#4813=DIRECTION('center_axis',(0.,-1.,0.));
#4814=DIRECTION('ref_axis',(0.965748659616483,0.,-0.259479337229319));
#4815=DIRECTION('',(0.,1.,0.));
#4816=DIRECTION('',(0.,1.,0.));
#4817=DIRECTION('center_axis',(1.,0.,0.));
#4818=DIRECTION('ref_axis',(0.,0.,-1.));
#4819=DIRECTION('',(0.,0.,1.));
#4820=DIRECTION('center_axis',(0.,1.,0.));
#4821=DIRECTION('ref_axis',(-1.,0.,-1.85962356624686E-14));
#4822=DIRECTION('center_axis',(0.,-1.,0.));
#4823=DIRECTION('ref_axis',(-1.,0.,-1.85962356624686E-14));
#4824=DIRECTION('',(0.,1.,0.));
#4825=DIRECTION('center_axis',(0.,1.,0.));
#4826=DIRECTION('ref_axis',(-0.965748659616478,0.,-0.259479337229339));
#4827=DIRECTION('center_axis',(0.,-1.,0.));
#4828=DIRECTION('ref_axis',(-0.965748659616478,0.,-0.259479337229339));
#4829=DIRECTION('center_axis',(1.,0.,0.));
#4830=DIRECTION('ref_axis',(0.,1.,0.));
#4831=DIRECTION('',(0.,1.,0.));
#4832=DIRECTION('',(0.,0.,1.));
#4833=DIRECTION('',(0.,-1.,0.));
#4834=DIRECTION('',(0.,0.,1.));
#4835=DIRECTION('center_axis',(0.,1.,0.));
#4836=DIRECTION('ref_axis',(-1.,0.,0.));
#4837=DIRECTION('',(-1.,0.,0.));
#4838=DIRECTION('',(0.,0.,1.));
#4839=DIRECTION('',(-1.,0.,0.));
#4840=DIRECTION('center_axis',(0.,0.,1.));
#4841=DIRECTION('ref_axis',(1.,0.,0.));
#4842=DIRECTION('center_axis',(0.,1.,0.));
#4843=DIRECTION('ref_axis',(-1.,0.,0.));
#4844=DIRECTION('',(-1.,0.,0.));
#4845=DIRECTION('',(0.,0.,1.));
#4846=DIRECTION('',(-1.,0.,0.));
#4847=DIRECTION('',(0.,0.,1.));
#4848=DIRECTION('center_axis',(0.,0.,1.));
#4849=DIRECTION('ref_axis',(0.,-1.,0.));
#4850=DIRECTION('center_axis',(0.,0.,-1.));
#4851=DIRECTION('ref_axis',(0.,-1.,0.));
#4852=DIRECTION('center_axis',(0.,0.,-1.));
#4853=DIRECTION('ref_axis',(0.,-1.,0.));
#4854=DIRECTION('',(0.,0.,1.));
#4855=DIRECTION('center_axis',(0.,-1.,0.));
#4856=DIRECTION('ref_axis',(1.,0.,0.));
#4857=DIRECTION('',(1.,0.,0.));
#4858=DIRECTION('',(1.,0.,0.));
#4859=DIRECTION('',(0.,0.,1.));
#4860=DIRECTION('center_axis',(0.,0.,1.));
#4861=DIRECTION('ref_axis',(0.,1.,0.));
#4862=DIRECTION('center_axis',(0.,0.,-1.));
#4863=DIRECTION('ref_axis',(0.,1.,0.));
#4864=DIRECTION('center_axis',(0.,0.,-1.));
#4865=DIRECTION('ref_axis',(0.,1.,0.));
#4866=DIRECTION('center_axis',(0.,1.,0.));
#4867=DIRECTION('ref_axis',(-1.,0.,0.));
#4868=DIRECTION('',(-1.,0.,0.));
#4869=DIRECTION('',(0.,0.,1.));
#4870=DIRECTION('',(-1.,0.,0.));
#4871=DIRECTION('',(0.,0.,1.));
#4872=DIRECTION('center_axis',(0.,0.,1.));
#4873=DIRECTION('ref_axis',(0.,-1.,0.));
#4874=DIRECTION('center_axis',(0.,0.,-1.));
#4875=DIRECTION('ref_axis',(0.,-1.,0.));
#4876=DIRECTION('center_axis',(0.,0.,-1.));
#4877=DIRECTION('ref_axis',(0.,-1.,0.));
#4878=DIRECTION('',(0.,0.,1.));
#4879=DIRECTION('center_axis',(0.,-1.,0.));
#4880=DIRECTION('ref_axis',(1.,0.,0.));
#4881=DIRECTION('',(1.,0.,0.));
#4882=DIRECTION('',(1.,0.,0.));
#4883=DIRECTION('',(0.,0.,1.));
#4884=DIRECTION('center_axis',(0.,0.,1.));
#4885=DIRECTION('ref_axis',(0.,1.,0.));
#4886=DIRECTION('center_axis',(0.,0.,-1.));
#4887=DIRECTION('ref_axis',(0.,1.,0.));
#4888=DIRECTION('center_axis',(0.,0.,-1.));
#4889=DIRECTION('ref_axis',(0.,1.,0.));
#4890=DIRECTION('center_axis',(-1.,-3.51417407375166E-16,0.));
#4891=DIRECTION('ref_axis',(3.51417407375166E-16,-1.,0.));
#4892=DIRECTION('',(0.,-1.,0.));
#4893=DIRECTION('',(0.,0.,1.));
#4894=DIRECTION('',(3.51417407375166E-16,-1.,0.));
#4895=DIRECTION('center_axis',(0.,0.,1.));
#4896=DIRECTION('ref_axis',(3.55271367880049E-15,-1.,0.));
#4897=DIRECTION('center_axis',(0.,0.,1.));
#4898=DIRECTION('ref_axis',(3.55271367880049E-15,-1.,0.));
#4899=DIRECTION('center_axis',(0.,0.,1.));
#4900=DIRECTION('ref_axis',(3.55271367880049E-15,-1.,0.));
#4901=DIRECTION('',(0.,0.,1.));
#4902=DIRECTION('center_axis',(-2.36032074788338E-16,-1.,0.));
#4903=DIRECTION('ref_axis',(1.,-2.36032074788338E-16,0.));
#4904=DIRECTION('',(-1.,2.36032074788338E-16,0.));
#4905=DIRECTION('',(1.,-2.36032074788338E-16,0.));
#4906=DIRECTION('',(0.,0.,1.));
#4907=DIRECTION('center_axis',(0.,0.,1.));
#4908=DIRECTION('ref_axis',(-1.,0.,0.));
#4909=DIRECTION('center_axis',(0.,0.,1.));
#4910=DIRECTION('ref_axis',(-1.,0.,0.));
#4911=DIRECTION('center_axis',(0.,0.,1.));
#4912=DIRECTION('ref_axis',(-1.,0.,0.));
#4913=DIRECTION('center_axis',(0.,0.,1.));
#4914=DIRECTION('ref_axis',(1.,0.,0.));
#4915=DIRECTION('center_axis',(0.,0.,1.));
#4916=DIRECTION('ref_axis',(1.,0.,0.));
#5815=CARTESIAN_POINT('',(0.,0.,0.));
#5816=CARTESIAN_POINT('Origin',(24.7143466872546,-3.13165946910082,-0.395297377936459));
#5817=CARTESIAN_POINT('',(24.7143466872546,-3.63165946910083,1.30603779103116));
#5818=CARTESIAN_POINT('Origin',(24.7143466872546,-3.63165946910082,-0.395297377936459));
#5819=CARTESIAN_POINT('',(24.7143466872546,-3.13165946910082,1.80603779103116));
#5820=CARTESIAN_POINT('Origin',(24.7143466872546,-3.13165946910082,1.30603779103116));
#5821=CARTESIAN_POINT('Origin',(24.7143466872546,-3.13165946910082,-0.395297377936459));
#5822=CARTESIAN_POINT('Origin',(24.7143466872546,-3.63165946910082,-0.395297377936459));
#5823=CARTESIAN_POINT('Origin',(37.3390884548007,-3.13165946910082,-0.451167579126729));
#5824=CARTESIAN_POINT('',(37.3390884548007,-3.63165946910083,1.30858121201868));
#5825=CARTESIAN_POINT('Origin',(37.3390884548007,-3.63165946910082,-0.451167579126729));
#5826=CARTESIAN_POINT('',(37.3390884548007,-3.13165946910082,1.80858121201868));
#5827=CARTESIAN_POINT('Origin',(37.3390884548007,-3.13165946910082,1.30858121201868));
#5828=CARTESIAN_POINT('Origin',(37.3390884548007,-3.13165946910082,-0.451167579126729));
#5829=CARTESIAN_POINT('Origin',(37.3390884548007,-3.63165946910082,-0.451167579126729));
#5830=CARTESIAN_POINT('Origin',(25.1607982446856,-4.63165946910082,-5.));
#5831=CARTESIAN_POINT('',(19.2071026744088,-4.63165946910082,-6.5));
#5832=CARTESIAN_POINT('',(19.8239560216472,-3.13165946910082,-5.));
#5833=CARTESIAN_POINT('Origin',(19.8239560216472,-4.63165946910082,-5.));
#5834=CARTESIAN_POINT('',(43.0218849555161,-4.63165946910082,-6.5));
#5835=CARTESIAN_POINT('',(25.1607982446856,-4.63165946910082,-6.5));
#5836=CARTESIAN_POINT('',(42.4050316082777,-3.13165946910082,-5.));
#5837=CARTESIAN_POINT('Origin',(42.4050316082777,-4.63165946910082,-5.));
#5838=CARTESIAN_POINT('',(25.1607982446856,-3.13165946910082,-5.));
#5839=CARTESIAN_POINT('Origin',(19.2071026744088,-3.13165946910082,-8.5));
#5840=CARTESIAN_POINT('',(40.0215468039921,-3.13165946910082,0.79591117148755));
#5841=CARTESIAN_POINT('',(41.6512074608448,-3.13165946910082,-3.16692861243009));
#5842=CARTESIAN_POINT('',(37.4782084817555,-3.13165946910082,2.5));
#5843=CARTESIAN_POINT('Origin',(37.4782084817555,-3.13165946910082,-0.25));
#5844=CARTESIAN_POINT('',(37.2590007645168,-3.13165946910082,2.5));
#5845=CARTESIAN_POINT('',(19.2071026744088,-3.13165946910082,2.5));
#5846=CARTESIAN_POINT('',(34.7590007645168,-3.13165946910082,0.));
#5847=CARTESIAN_POINT('Origin',(37.2590007645168,-3.13165946910082,0.));
#5848=CARTESIAN_POINT('',(34.7590007645168,-3.13165946910082,-0.758936728277321));
#5849=CARTESIAN_POINT('',(34.7590007645168,-3.13165946910082,-3.));
#5850=CARTESIAN_POINT('',(34.6904980837498,-3.13165946910082,-1.277895402736));
#5851=CARTESIAN_POINT('Origin',(32.7590007645165,-3.13165946910082,-0.758936728277284));
#5852=CARTESIAN_POINT('',(27.5384895461752,-3.13165946910082,-1.277895402736));
#5853=CARTESIAN_POINT('Origin',(31.1144938149625,-3.13165946910082,-0.317087216926334));
#5854=CARTESIAN_POINT('',(27.4699868654081,-3.13165946910082,-0.758936728277321));
#5855=CARTESIAN_POINT('Origin',(29.4699868654084,-3.13165946910082,-0.758936728277284));
#5856=CARTESIAN_POINT('',(27.4699868654081,-3.13165946910082,0.));
#5857=CARTESIAN_POINT('',(27.4699868654081,-3.13165946910082,-4.62946836413866));
#5858=CARTESIAN_POINT('',(24.9699868654081,-3.13165946910082,2.5));
#5859=CARTESIAN_POINT('Origin',(24.9699868654081,-3.13165946910082,0.));
#5860=CARTESIAN_POINT('',(24.7507791481694,-3.13165946910082,2.5));
#5861=CARTESIAN_POINT('',(19.2071026744088,-3.13165946910082,2.5));
#5862=CARTESIAN_POINT('',(22.2074408259328,-3.13165946910082,0.795911171487552));
#5863=CARTESIAN_POINT('Origin',(24.7507791481694,-3.13165946910082,-0.25));
#5864=CARTESIAN_POINT('',(20.7059131671521,-3.13165946910082,-2.85534807555141));
#5865=CARTESIAN_POINT('Origin',(37.2590007645168,-2.75665946910082,0.));
#5866=CARTESIAN_POINT('',(37.2590007645168,-1.63165946910082,2.5));
#5867=CARTESIAN_POINT('',(37.2590007645168,-2.75665946910082,2.5));
#5868=CARTESIAN_POINT('',(34.7590007645168,-1.63165946910082,0.));
#5869=CARTESIAN_POINT('Origin',(37.2590007645168,-1.63165946910082,0.));
#5870=CARTESIAN_POINT('',(34.7590007645168,-2.75665946910082,0.));
#5871=CARTESIAN_POINT('Origin',(31.1144938149625,-2.38165946910082,2.5));
#5872=CARTESIAN_POINT('',(37.4782084817555,-1.63165946910082,2.5));
#5873=CARTESIAN_POINT('',(37.4782084817555,-2.75665946910082,2.5));
#5874=CARTESIAN_POINT('',(43.0218849555161,-1.63165946910082,2.5));
#5875=CARTESIAN_POINT('Origin',(24.9699868654081,-2.75665946910082,0.));
#5876=CARTESIAN_POINT('',(27.4699868654081,-1.63165946910082,0.));
#5877=CARTESIAN_POINT('',(24.9699868654081,-1.63165946910082,2.5));
#5878=CARTESIAN_POINT('Origin',(24.9699868654081,-1.63165946910082,0.));
#5879=CARTESIAN_POINT('',(24.9699868654081,-2.75665946910082,2.5));
#5880=CARTESIAN_POINT('',(27.4699868654081,-2.75665946910082,0.));
#5881=CARTESIAN_POINT('Origin',(27.4699868654081,-3.13165946910082,-0.758936728277321));
#5882=CARTESIAN_POINT('',(27.4699868654081,-1.63165946910082,-0.758936728277321));
#5883=CARTESIAN_POINT('',(27.4699868654081,-3.13165946910082,-0.758936728277321));
#5884=CARTESIAN_POINT('',(27.4699868654081,-1.63165946910082,-4.62946836413866));
#5885=CARTESIAN_POINT('Origin',(37.4782084817555,-2.75665946910082,-0.25));
#5886=CARTESIAN_POINT('',(40.0215468039921,-1.63165946910082,0.795911171487551));
#5887=CARTESIAN_POINT('Origin',(37.4782084817555,-1.63165946910082,-0.25));
#5888=CARTESIAN_POINT('',(40.0215468039921,-2.75665946910082,0.795911171487553));
#5889=CARTESIAN_POINT('Origin',(43.0218849555161,-3.13165946910082,-6.5));
#5890=CARTESIAN_POINT('',(43.0218849555161,-1.63165946910082,-6.5));
#5891=CARTESIAN_POINT('',(43.0218849555161,-3.13165946910082,-6.5));
#5892=CARTESIAN_POINT('',(43.373634504488,-1.63165946910082,-7.35534807555141));
#5893=CARTESIAN_POINT('Origin',(24.7507791481694,-2.75665946910082,-0.25));
#5894=CARTESIAN_POINT('',(24.7507791481694,-1.63165946910082,2.5));
#5895=CARTESIAN_POINT('',(24.7507791481694,-2.75665946910082,2.5));
#5896=CARTESIAN_POINT('',(22.2074408259328,-1.63165946910082,0.795911171487552));
#5897=CARTESIAN_POINT('Origin',(24.7507791481694,-1.63165946910082,-0.25));
#5898=CARTESIAN_POINT('',(22.2074408259328,-2.75665946910082,0.795911171487551));
#5899=CARTESIAN_POINT('Origin',(22.9082227578391,-3.13165946910082,2.5));
#5900=CARTESIAN_POINT('',(19.2071026744088,-1.63165946910082,-6.5));
#5901=CARTESIAN_POINT('',(22.4283402107953,-1.63165946910082,1.3330713875699));
#5902=CARTESIAN_POINT('',(19.2071026744088,-9.4502026108178,-6.5));
#5903=CARTESIAN_POINT('Origin',(32.7590007645165,-3.13165946910082,-0.758936728277284));
#5904=CARTESIAN_POINT('',(34.6904980837498,-1.63165946910082,-1.277895402736));
#5905=CARTESIAN_POINT('',(34.7590007645168,-1.63165946910082,-0.758936728277321));
#5906=CARTESIAN_POINT('Origin',(32.7590007645165,-1.63165946910082,-0.758936728277284));
#5907=CARTESIAN_POINT('',(34.6904980837498,-3.13165946910082,-1.277895402736));
#5908=CARTESIAN_POINT('',(34.7590007645168,-3.13165946910082,-0.758936728277321));
#5909=CARTESIAN_POINT('Origin',(34.7590007645168,-3.13165946910082,2.5));
#5910=CARTESIAN_POINT('',(34.7590007645168,-1.63165946910082,-3.));
#5911=CARTESIAN_POINT('Origin',(29.4699868654084,-3.13165946910082,-0.758936728277284));
#5912=CARTESIAN_POINT('',(27.5384895461752,-1.63165946910082,-1.277895402736));
#5913=CARTESIAN_POINT('Origin',(29.4699868654084,-1.63165946910082,-0.758936728277284));
#5914=CARTESIAN_POINT('',(27.5384895461752,-3.13165946910082,-1.277895402736));
#5915=CARTESIAN_POINT('Origin',(31.1144938149625,-3.13165946910082,-0.317087216926334));
#5916=CARTESIAN_POINT('Origin',(31.1144938149625,-1.63165946910082,-0.317087216926334));
#5917=CARTESIAN_POINT('Origin',(43.0218849555161,-9.4502026108178,-8.5));
#5918=CARTESIAN_POINT('',(43.0218849555161,-9.4502026108178,-6.5));
#5919=CARTESIAN_POINT('',(43.0218849555161,-3.13165946910082,-6.5));
#5920=CARTESIAN_POINT('',(43.0218849555161,-9.4502026108178,-8.5));
#5921=CARTESIAN_POINT('',(43.0218849555161,-9.4502026108178,-8.5));
#5922=CARTESIAN_POINT('',(43.0218849555161,-1.63165946910082,-8.5));
#5923=CARTESIAN_POINT('',(43.0218849555161,-3.13165946910082,-8.5));
#5924=CARTESIAN_POINT('',(43.0218849555161,-1.63165946910082,-8.5));
#5925=CARTESIAN_POINT('Origin',(43.0218849555161,-1.63165946910082,-8.5));
#5926=CARTESIAN_POINT('',(19.2071026744088,-1.63165946910082,-8.5));
#5927=CARTESIAN_POINT('',(43.0218849555161,-1.63165946910082,-8.5));
#5928=CARTESIAN_POINT('',(19.2071026744088,-1.63165946910082,-8.5));
#5929=CARTESIAN_POINT('',(43.0218849555161,-1.63165946910082,2.5));
#5930=CARTESIAN_POINT('Origin',(31.1144938149625,-2.38165946910082,2.5));
#5931=CARTESIAN_POINT('Origin',(38.9466240721952,-10.3406188648021,-8.5));
#5932=CARTESIAN_POINT('',(38.9466240721952,-10.3406188648021,-8.5));
#5933=CARTESIAN_POINT('',(36.8121029357457,-10.3406188648021,-8.5));
#5934=CARTESIAN_POINT('',(36.8121029357457,-10.3406188648021,-8.5));
#5935=CARTESIAN_POINT('',(36.8121029357457,-10.3406188648021,-6.5));
#5936=CARTESIAN_POINT('',(36.8121029357457,-10.3406188648021,-8.5));
#5937=CARTESIAN_POINT('',(38.9466240721952,-10.3406188648021,-6.5));
#5938=CARTESIAN_POINT('',(36.8121029357457,-10.3406188648021,-6.5));
#5939=CARTESIAN_POINT('',(38.9466240721952,-10.3406188648021,-8.5));
#5940=CARTESIAN_POINT('Origin',(38.9466240721952,-8.04398219900198,-8.5));
#5941=CARTESIAN_POINT('',(38.9466240721952,-5.74734553320186,-8.5));
#5942=CARTESIAN_POINT('Origin',(38.9466240721952,-8.04398219900198,-8.5));
#5943=CARTESIAN_POINT('',(38.9466240721952,-5.74734553320186,-6.5));
#5944=CARTESIAN_POINT('Origin',(38.9466240721952,-8.04398219900198,-6.5));
#5945=CARTESIAN_POINT('',(38.9466240721952,-5.74734553320186,-8.5));
#5946=CARTESIAN_POINT('Origin',(36.8121029357457,-5.74734553320186,-8.5));
#5947=CARTESIAN_POINT('',(36.8121029357457,-5.74734553320186,-8.5));
#5948=CARTESIAN_POINT('',(38.9466240721952,-5.74734553320186,-8.5));
#5949=CARTESIAN_POINT('',(36.8121029357457,-5.74734553320186,-6.5));
#5950=CARTESIAN_POINT('',(38.9466240721952,-5.74734553320186,-6.5));
#5951=CARTESIAN_POINT('',(36.8121029357457,-5.74734553320186,-8.5));
#5952=CARTESIAN_POINT('Origin',(36.8121029357457,-8.04398219900198,-8.5));
#5953=CARTESIAN_POINT('Origin',(36.8121029357457,-8.04398219900198,-8.5));
#5954=CARTESIAN_POINT('Origin',(36.8121029357457,-8.04398219900198,-6.5));
#5955=CARTESIAN_POINT('Origin',(25.4466240721952,-10.3406188648021,-8.5));
#5956=CARTESIAN_POINT('',(25.4466240721952,-10.3406188648021,-8.5));
#5957=CARTESIAN_POINT('',(23.3121029357457,-10.3406188648021,-8.5));
#5958=CARTESIAN_POINT('',(23.3121029357457,-10.3406188648021,-8.5));
#5959=CARTESIAN_POINT('',(23.3121029357457,-10.3406188648021,-6.5));
#5960=CARTESIAN_POINT('',(23.3121029357457,-10.3406188648021,-8.5));
#5961=CARTESIAN_POINT('',(25.4466240721952,-10.3406188648021,-6.5));
#5962=CARTESIAN_POINT('',(23.3121029357457,-10.3406188648021,-6.5));
#5963=CARTESIAN_POINT('',(25.4466240721952,-10.3406188648021,-8.5));
#5964=CARTESIAN_POINT('Origin',(25.4466240721952,-8.04398219900198,-8.5));
#5965=CARTESIAN_POINT('',(25.4466240721952,-5.74734553320186,-8.5));
#5966=CARTESIAN_POINT('Origin',(25.4466240721952,-8.04398219900198,-8.5));
#5967=CARTESIAN_POINT('',(25.4466240721952,-5.74734553320186,-6.5));
#5968=CARTESIAN_POINT('Origin',(25.4466240721952,-8.04398219900198,-6.5));
#5969=CARTESIAN_POINT('',(25.4466240721952,-5.74734553320186,-8.5));
#5970=CARTESIAN_POINT('Origin',(23.3121029357457,-5.74734553320186,-8.5));
#5971=CARTESIAN_POINT('',(23.3121029357457,-5.74734553320186,-8.5));
#5972=CARTESIAN_POINT('',(25.4466240721952,-5.74734553320186,-8.5));
#5973=CARTESIAN_POINT('',(23.3121029357457,-5.74734553320186,-6.5));
#5974=CARTESIAN_POINT('',(25.4466240721952,-5.74734553320186,-6.5));
#5975=CARTESIAN_POINT('',(23.3121029357457,-5.74734553320186,-8.5));
#5976=CARTESIAN_POINT('Origin',(23.3121029357457,-8.04398219900198,-8.5));
#5977=CARTESIAN_POINT('Origin',(23.3121029357457,-8.04398219900198,-8.5));
#5978=CARTESIAN_POINT('Origin',(23.3121029357457,-8.04398219900198,-6.5));
#5979=CARTESIAN_POINT('Origin',(19.2071026744088,-3.13165946910082,-8.5));
#5980=CARTESIAN_POINT('',(19.2071026744088,-9.4502026108178,-8.5));
#5981=CARTESIAN_POINT('',(19.2071026744088,-1.63165946910082,-8.5));
#5982=CARTESIAN_POINT('',(19.2071026744088,-9.4502026108178,-6.5));
#5983=CARTESIAN_POINT('',(19.2071026744088,-9.4502026108178,-8.5));
#5984=CARTESIAN_POINT('',(19.2071026744088,-9.4502026108178,-6.5));
#5985=CARTESIAN_POINT('Origin',(40.5218849555161,-9.45020261081779,-8.5));
#5986=CARTESIAN_POINT('',(40.5218849555161,-11.9502026108178,-8.5));
#5987=CARTESIAN_POINT('Origin',(40.5218849555161,-9.45020261081779,-8.5));
#5988=CARTESIAN_POINT('',(40.5218849555161,-11.9502026108178,-6.5));
#5989=CARTESIAN_POINT('Origin',(40.5218849555161,-9.45020261081779,-6.5));
#5990=CARTESIAN_POINT('',(40.5218849555161,-11.9502026108178,-8.5));
#5991=CARTESIAN_POINT('Origin',(21.7071026744088,-11.9502026108178,-8.5));
#5992=CARTESIAN_POINT('',(21.7071026744088,-11.9502026108178,-8.5));
#5993=CARTESIAN_POINT('',(40.5218849555161,-11.9502026108178,-8.5));
#5994=CARTESIAN_POINT('',(21.7071026744088,-11.9502026108178,-6.5));
#5995=CARTESIAN_POINT('',(40.5218849555161,-11.9502026108178,-6.5));
#5996=CARTESIAN_POINT('',(21.7071026744088,-11.9502026108178,-8.5));
#5997=CARTESIAN_POINT('Origin',(21.7071026744088,-9.4502026108178,-8.5));
#5998=CARTESIAN_POINT('Origin',(21.7071026744088,-9.4502026108178,-8.5));
#5999=CARTESIAN_POINT('Origin',(21.7071026744088,-9.4502026108178,-6.5));
#6000=CARTESIAN_POINT('Origin',(31.1144938149625,-7.54093103995931,-6.5));
#6001=CARTESIAN_POINT('Origin',(31.1144938149625,-7.54093103995931,-8.5));
#23558=UNCERTAINTY_MEASURE_WITH_UNIT(LENGTH_MEASURE(0.01),#23578,
'DISTANCE_ACCURACY_VALUE',
'Maximum model space distance between geometric entities at asserted c
onnectivities');
#23566=UNCERTAINTY_MEASURE_WITH_UNIT(LENGTH_MEASURE(0.01),#23578,
'DISTANCE_ACCURACY_VALUE',
'Maximum model space distance between geometric entities at asserted c
onnectivities');
#23569=(
GEOMETRIC_REPRESENTATION_CONTEXT(3)
GLOBAL_UNCERTAINTY_ASSIGNED_CONTEXT((#23558))
GLOBAL_UNIT_ASSIGNED_CONTEXT((#23578,#23580,#23581))
REPRESENTATION_CONTEXT('','3D')
);
#23577=(
GEOMETRIC_REPRESENTATION_CONTEXT(3)
GLOBAL_UNCERTAINTY_ASSIGNED_CONTEXT((#23566))
GLOBAL_UNIT_ASSIGNED_CONTEXT((#23578,#23580,#23581))
REPRESENTATION_CONTEXT('','3D')
);
#23578=(
LENGTH_UNIT()
NAMED_UNIT(*)
SI_UNIT(.MILLI.,.METRE.)
);
#23580=(
NAMED_UNIT(*)
PLANE_ANGLE_UNIT()
SI_UNIT($,.RADIAN.)
);
#23581=(
NAMED_UNIT(*)
SI_UNIT($,.STERADIAN.)
SOLID_ANGLE_UNIT()
);
#23584=SHAPE_DEFINITION_REPRESENTATION(#23594,#23613);
#23594=PRODUCT_DEFINITION_SHAPE('',$,#23624);
#23613=SHAPE_REPRESENTATION('',(#4284),#23569);
#23621=PRODUCT_DEFINITION_CONTEXT('part definition',#23653,'design');
#23624=PRODUCT_DEFINITION('Base_Left','Base_Left',#23634,#23621);
#23634=PRODUCT_DEFINITION_FORMATION('',$,#23657);
#23653=APPLICATION_CONTEXT(
'Core Data for Automotive Mechanical Design Process');
#23654=PRODUCT_CONTEXT('part definition',#23653,'mechanical');
#23657=PRODUCT('Base_Left','Base_Left',$,(#23654));
#23666=PRESENTATION_STYLE_ASSIGNMENT((#23671));
#23671=SURFACE_STYLE_USAGE(.BOTH.,#23676);
#23676=SURFACE_SIDE_STYLE('',(#23681));
#23681=SURFACE_STYLE_FILL_AREA(#23686);
#23686=FILL_AREA_STYLE('Opaque(210,210,210)',(#23691));
#23691=FILL_AREA_STYLE_COLOUR('Opaque(210,210,210)',#23696);
#23696=COLOUR_RGB('Opaque(210,210,210)', 0.09019608, 0.27058824, 0.51372549);
ENDSEC;
END-ISO-10303-21;
